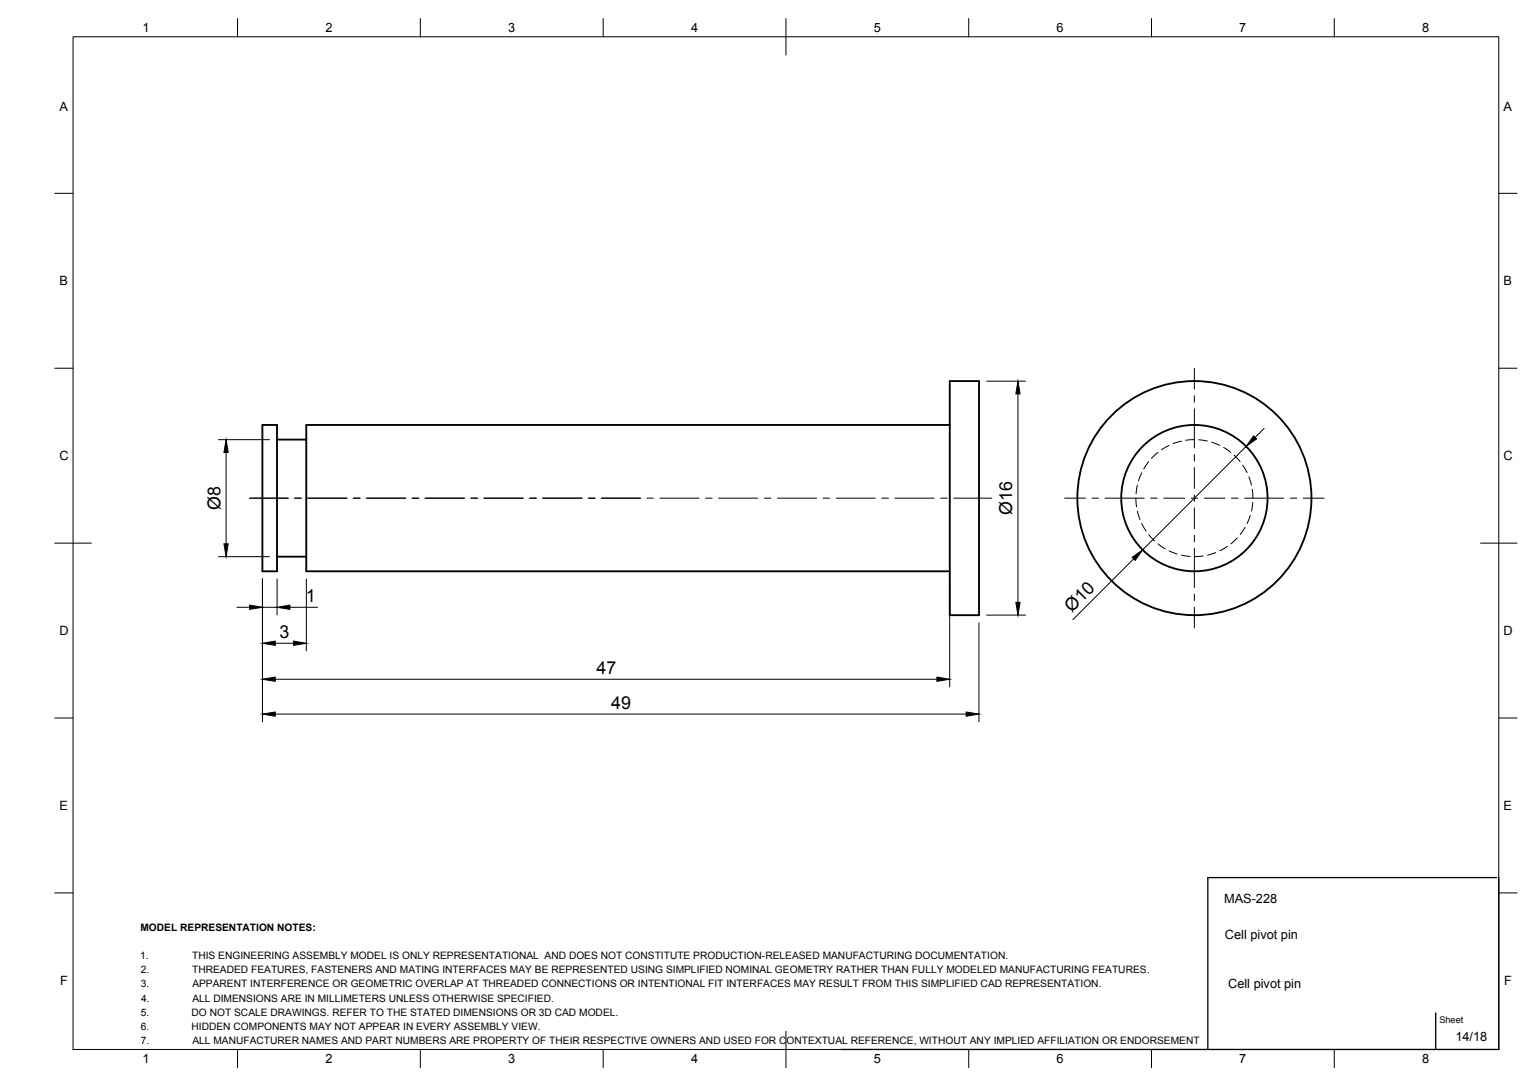
ISO-10303-21;
HEADER;
/* Generated by software containing ST-Developer
 * from STEP Tools, Inc. (www.steptools.com) 
 */

FILE_DESCRIPTION(
/* description */ ('Independent Peaucellier-Lipkin straight-line linkage. Radius arms 100
 mm, inversion-cell links 60 mm, crank radius and fixed-pivot spacing 
32 mm. Inversion constant 6400 mm squared, nominal output straight lin
e X=100 mm. Overhead bearing bridge clears the layered moving links. N
o accuracy or load rating assigned.'),
/* implementation_level */ '2;1');

FILE_NAME(
/* name */ 'Cell pivot pin.step',
/* time_stamp */ '2026-11-09T18:06:16-08:00',
/* author */ (''),
/* organization */ (''),
/* preprocessor_version */ 'ST-DEVELOPER v20.2',
/* originating_system */ 'Autodesk Translation Framework v15.17.0.0',
/* authorisation */ '');

FILE_SCHEMA (('AUTOMOTIVE_DESIGN { 1 0 10303 214 3 1 1 }'));
ENDSEC;

DATA;
#10=MECHANICAL_DESIGN_GEOMETRIC_PRESENTATION_REPRESENTATION('',(#295),#3581);
#261=SHAPE_REPRESENTATION_RELATIONSHIP('SRR','None',#3695,#278);
#278=ADVANCED_BREP_SHAPE_REPRESENTATION('',(#312),#3577);
#295=STYLED_ITEM('',(#3782),#312);
#312=MANIFOLD_SOLID_BREP('Body1',#1881);
#357=FACE_BOUND('',#667,.T.);
#358=FACE_BOUND('',#669,.T.);
#359=FACE_BOUND('',#672,.T.);
#412=PLANE('',#2257);
#413=PLANE('',#2259);
#414=PLANE('',#2263);
#415=PLANE('',#2268);
#416=PLANE('',#2270);
#513=FACE_OUTER_BOUND('',#665,.T.);
#514=FACE_OUTER_BOUND('',#666,.T.);
#515=FACE_OUTER_BOUND('',#668,.T.);
#516=FACE_OUTER_BOUND('',#670,.T.);
#517=FACE_OUTER_BOUND('',#671,.T.);
#518=FACE_OUTER_BOUND('',#673,.T.);
#519=FACE_OUTER_BOUND('',#674,.T.);
#520=FACE_OUTER_BOUND('',#675,.T.);
#521=FACE_OUTER_BOUND('',#676,.T.);
#665=EDGE_LOOP('',(#1636,#1637,#1638,#1639));
#666=EDGE_LOOP('',(#1640));
#667=EDGE_LOOP('',(#1641));
#668=EDGE_LOOP('',(#1642));
#669=EDGE_LOOP('',(#1643));
#670=EDGE_LOOP('',(#1644,#1645,#1646,#1647));
#671=EDGE_LOOP('',(#1648));
#672=EDGE_LOOP('',(#1649));
#673=EDGE_LOOP('',(#1650,#1651,#1652,#1653));
#674=EDGE_LOOP('',(#1654));
#675=EDGE_LOOP('',(#1655,#1656,#1657,#1658));
#676=EDGE_LOOP('',(#1659));
#777=LINE('',#3403,#875);
#778=LINE('',#3414,#876);
#779=LINE('',#3422,#877);
#780=LINE('',#3426,#878);
#875=VECTOR('',#2807,4.);
#876=VECTOR('',#2822,5.);
#877=VECTOR('',#2831,8.);
#878=VECTOR('',#2838,5.);
#969=CIRCLE('',#2255,4.);
#970=CIRCLE('',#2256,4.);
#971=CIRCLE('',#2258,5.);
#972=CIRCLE('',#2260,5.);
#973=CIRCLE('',#2262,5.);
#974=CIRCLE('',#2264,8.);
#975=CIRCLE('',#2265,5.);
#976=CIRCLE('',#2267,8.);
#1096=VERTEX_POINT('',#3400);
#1097=VERTEX_POINT('',#3402);
#1098=VERTEX_POINT('',#3406);
#1099=VERTEX_POINT('',#3409);
#1100=VERTEX_POINT('',#3412);
#1101=VERTEX_POINT('',#3416);
#1102=VERTEX_POINT('',#3418);
#1103=VERTEX_POINT('',#3421);
#1280=EDGE_CURVE('',#1096,#1096,#969,.T.);
#1281=EDGE_CURVE('',#1096,#1097,#777,.T.);
#1282=EDGE_CURVE('',#1097,#1097,#970,.T.);
#1283=EDGE_CURVE('',#1098,#1098,#971,.T.);
#1284=EDGE_CURVE('',#1099,#1099,#972,.T.);
#1285=EDGE_CURVE('',#1100,#1100,#973,.T.);
#1286=EDGE_CURVE('',#1100,#1099,#778,.T.);
#1287=EDGE_CURVE('',#1101,#1101,#974,.T.);
#1288=EDGE_CURVE('',#1102,#1102,#975,.T.);
#1289=EDGE_CURVE('',#1101,#1103,#779,.T.);
#1290=EDGE_CURVE('',#1103,#1103,#976,.T.);
#1291=EDGE_CURVE('',#1098,#1102,#780,.T.);
#1636=ORIENTED_EDGE('',*,*,#1280,.T.);
#1637=ORIENTED_EDGE('',*,*,#1281,.T.);
#1638=ORIENTED_EDGE('',*,*,#1282,.F.);
#1639=ORIENTED_EDGE('',*,*,#1281,.F.);
#1640=ORIENTED_EDGE('',*,*,#1283,.F.);
#1641=ORIENTED_EDGE('',*,*,#1280,.F.);
#1642=ORIENTED_EDGE('',*,*,#1284,.F.);
#1643=ORIENTED_EDGE('',*,*,#1282,.T.);
#1644=ORIENTED_EDGE('',*,*,#1285,.F.);
#1645=ORIENTED_EDGE('',*,*,#1286,.T.);
#1646=ORIENTED_EDGE('',*,*,#1284,.T.);
#1647=ORIENTED_EDGE('',*,*,#1286,.F.);
#1648=ORIENTED_EDGE('',*,*,#1287,.T.);
#1649=ORIENTED_EDGE('',*,*,#1288,.F.);
#1650=ORIENTED_EDGE('',*,*,#1287,.F.);
#1651=ORIENTED_EDGE('',*,*,#1289,.T.);
#1652=ORIENTED_EDGE('',*,*,#1290,.T.);
#1653=ORIENTED_EDGE('',*,*,#1289,.F.);
#1654=ORIENTED_EDGE('',*,*,#1290,.F.);
#1655=ORIENTED_EDGE('',*,*,#1283,.T.);
#1656=ORIENTED_EDGE('',*,*,#1291,.T.);
#1657=ORIENTED_EDGE('',*,*,#1288,.T.);
#1658=ORIENTED_EDGE('',*,*,#1291,.F.);
#1659=ORIENTED_EDGE('',*,*,#1285,.T.);
#1747=CYLINDRICAL_SURFACE('',#2254,4.);
#1748=CYLINDRICAL_SURFACE('',#2261,5.);
#1749=CYLINDRICAL_SURFACE('',#2266,8.);
#1750=CYLINDRICAL_SURFACE('',#2269,5.);
#1845=ADVANCED_FACE('',(#513),#1747,.T.);
#1846=ADVANCED_FACE('',(#514,#357),#412,.F.);
#1847=ADVANCED_FACE('',(#515,#358),#413,.F.);
#1848=ADVANCED_FACE('',(#516),#1748,.T.);
#1849=ADVANCED_FACE('',(#517,#359),#414,.T.);
#1850=ADVANCED_FACE('',(#518),#1749,.T.);
#1851=ADVANCED_FACE('',(#519),#415,.F.);
#1852=ADVANCED_FACE('',(#520),#1750,.T.);
#1853=ADVANCED_FACE('',(#521),#416,.T.);
#1881=CLOSED_SHELL('',(#1845,#1846,#1847,#1848,#1849,#1850,#1851,#1852,
#1853));
#2253=AXIS2_PLACEMENT_3D('',#3398,#2801,#2802);
#2254=AXIS2_PLACEMENT_3D('',#3399,#2803,#2804);
#2255=AXIS2_PLACEMENT_3D('',#3401,#2805,#2806);
#2256=AXIS2_PLACEMENT_3D('',#3404,#2808,#2809);
#2257=AXIS2_PLACEMENT_3D('',#3405,#2810,#2811);
#2258=AXIS2_PLACEMENT_3D('',#3407,#2812,#2813);
#2259=AXIS2_PLACEMENT_3D('',#3408,#2814,#2815);
#2260=AXIS2_PLACEMENT_3D('',#3410,#2816,#2817);
#2261=AXIS2_PLACEMENT_3D('',#3411,#2818,#2819);
#2262=AXIS2_PLACEMENT_3D('',#3413,#2820,#2821);
#2263=AXIS2_PLACEMENT_3D('',#3415,#2823,#2824);
#2264=AXIS2_PLACEMENT_3D('',#3417,#2825,#2826);
#2265=AXIS2_PLACEMENT_3D('',#3419,#2827,#2828);
#2266=AXIS2_PLACEMENT_3D('',#3420,#2829,#2830);
#2267=AXIS2_PLACEMENT_3D('',#3423,#2832,#2833);
#2268=AXIS2_PLACEMENT_3D('',#3424,#2834,#2835);
#2269=AXIS2_PLACEMENT_3D('',#3425,#2836,#2837);
#2270=AXIS2_PLACEMENT_3D('',#3427,#2839,#2840);
#2801=DIRECTION('axis',(0.,0.,1.));
#2802=DIRECTION('refdir',(1.,0.,0.));
#2803=DIRECTION('center_axis',(0.,0.,1.));
#2804=DIRECTION('ref_axis',(1.,0.,0.));
#2805=DIRECTION('center_axis',(0.,0.,1.));
#2806=DIRECTION('ref_axis',(1.,0.,0.));
#2807=DIRECTION('',(0.,0.,1.));
#2808=DIRECTION('center_axis',(0.,0.,1.));
#2809=DIRECTION('ref_axis',(1.,0.,0.));
#2810=DIRECTION('center_axis',(0.,0.,-1.));
#2811=DIRECTION('ref_axis',(-1.,0.,0.));
#2812=DIRECTION('center_axis',(0.,0.,-1.));
#2813=DIRECTION('ref_axis',(1.,0.,0.));
#2814=DIRECTION('center_axis',(0.,0.,1.));
#2815=DIRECTION('ref_axis',(1.,0.,0.));
#2816=DIRECTION('center_axis',(0.,0.,1.));
#2817=DIRECTION('ref_axis',(1.,0.,0.));
#2818=DIRECTION('center_axis',(0.,0.,1.));
#2819=DIRECTION('ref_axis',(1.,0.,0.));
#2820=DIRECTION('center_axis',(0.,0.,1.));
#2821=DIRECTION('ref_axis',(1.,0.,0.));
#2822=DIRECTION('',(0.,0.,-1.));
#2823=DIRECTION('center_axis',(0.,0.,1.));
#2824=DIRECTION('ref_axis',(1.,0.,0.));
#2825=DIRECTION('center_axis',(0.,0.,1.));
#2826=DIRECTION('ref_axis',(1.,0.,0.));
#2827=DIRECTION('center_axis',(0.,0.,1.));
#2828=DIRECTION('ref_axis',(1.,0.,0.));
#2829=DIRECTION('center_axis',(0.,0.,1.));
#2830=DIRECTION('ref_axis',(1.,0.,0.));
#2831=DIRECTION('',(0.,0.,-1.));
#2832=DIRECTION('center_axis',(0.,0.,1.));
#2833=DIRECTION('ref_axis',(1.,0.,0.));
#2834=DIRECTION('center_axis',(0.,0.,1.));
#2835=DIRECTION('ref_axis',(1.,0.,0.));
#2836=DIRECTION('center_axis',(0.,0.,1.));
#2837=DIRECTION('ref_axis',(1.,0.,0.));
#2838=DIRECTION('',(0.,0.,-1.));
#2839=DIRECTION('center_axis',(0.,0.,1.));
#2840=DIRECTION('ref_axis',(1.,0.,0.));
#3398=CARTESIAN_POINT('',(0.,0.,0.));
#3399=CARTESIAN_POINT('Origin',(0.,0.,45.));
#3400=CARTESIAN_POINT('',(-4.,-4.89858719658941E-16,44.));
#3401=CARTESIAN_POINT('Origin',(0.,0.,44.));
#3402=CARTESIAN_POINT('',(-4.,-4.89858719658941E-16,46.));
#3403=CARTESIAN_POINT('',(-4.,-4.89858719658941E-16,45.));
#3404=CARTESIAN_POINT('Origin',(0.,0.,46.));
#3405=CARTESIAN_POINT('Origin',(8.,0.,44.));
#3406=CARTESIAN_POINT('',(-5.,6.12323399573677E-16,44.));
#3407=CARTESIAN_POINT('Origin',(0.,0.,44.));
#3408=CARTESIAN_POINT('Origin',(4.,0.,46.));
#3409=CARTESIAN_POINT('',(-5.,-6.12323399573677E-16,46.));
#3410=CARTESIAN_POINT('Origin',(0.,0.,46.));
#3411=CARTESIAN_POINT('Origin',(0.,0.,0.));
#3412=CARTESIAN_POINT('',(-5.,-6.12323399573677E-16,47.));
#3413=CARTESIAN_POINT('Origin',(0.,0.,47.));
#3414=CARTESIAN_POINT('',(-5.,-6.12323399573677E-16,0.));
#3415=CARTESIAN_POINT('Origin',(0.,0.,0.));
#3416=CARTESIAN_POINT('',(-8.,-9.79717439317883E-16,0.));
#3417=CARTESIAN_POINT('Origin',(0.,0.,0.));
#3418=CARTESIAN_POINT('',(-5.,-6.12323399573677E-16,0.));
#3419=CARTESIAN_POINT('Origin',(0.,0.,0.));
#3420=CARTESIAN_POINT('Origin',(0.,0.,-2.));
#3421=CARTESIAN_POINT('',(-8.,-9.79717439317883E-16,-2.));
#3422=CARTESIAN_POINT('',(-8.,-9.79717439317883E-16,-2.));
#3423=CARTESIAN_POINT('Origin',(0.,0.,-2.));
#3424=CARTESIAN_POINT('Origin',(0.,0.,-2.));
#3425=CARTESIAN_POINT('Origin',(0.,0.,0.));
#3426=CARTESIAN_POINT('',(-5.,-6.12323399573677E-16,0.));
#3427=CARTESIAN_POINT('Origin',(0.,0.,47.));
#3558=UNCERTAINTY_MEASURE_WITH_UNIT(LENGTH_MEASURE(0.01),#3582,
'DISTANCE_ACCURACY_VALUE',
'Maximum model space distance between geometric entities at asserted c
onnectivities');
#3562=UNCERTAINTY_MEASURE_WITH_UNIT(LENGTH_MEASURE(0.01),#3582,
'DISTANCE_ACCURACY_VALUE',
'Maximum model space distance between geometric entities at asserted c
onnectivities');
#3577=(
GEOMETRIC_REPRESENTATION_CONTEXT(3)
GLOBAL_UNCERTAINTY_ASSIGNED_CONTEXT((#3558))
GLOBAL_UNIT_ASSIGNED_CONTEXT((#3582,#3584,#3585))
REPRESENTATION_CONTEXT('','3D')
);
#3581=(
GEOMETRIC_REPRESENTATION_CONTEXT(3)
GLOBAL_UNCERTAINTY_ASSIGNED_CONTEXT((#3562))
GLOBAL_UNIT_ASSIGNED_CONTEXT((#3582,#3584,#3585))
REPRESENTATION_CONTEXT('','3D')
);
#3582=(
LENGTH_UNIT()
NAMED_UNIT(*)
SI_UNIT(.MILLI.,.METRE.)
);
#3584=(
NAMED_UNIT(*)
PLANE_ANGLE_UNIT()
SI_UNIT($,.RADIAN.)
);
#3585=(
NAMED_UNIT(*)
SI_UNIT($,.STERADIAN.)
SOLID_ANGLE_UNIT()
);
#3600=SHAPE_DEFINITION_REPRESENTATION(#3618,#3695);
#3618=PRODUCT_DEFINITION_SHAPE('',$,#3714);
#3695=SHAPE_REPRESENTATION('',(#2253),#3577);
#3699=PRODUCT_DEFINITION_CONTEXT('part definition',#3755,'design');
#3714=PRODUCT_DEFINITION('Cell pivot pin','Cell pivot pin',#3732,#3699);
#3732=PRODUCT_DEFINITION_FORMATION('',$,#3771);
#3755=APPLICATION_CONTEXT(
'Core Data for Automotive Mechanical Design Process');
#3756=PRODUCT_CONTEXT('part definition',#3755,'mechanical');
#3771=PRODUCT('Cell pivot pin','Cell pivot pin',$,(#3756));
#3782=PRESENTATION_STYLE_ASSIGNMENT((#3795));
#3795=SURFACE_STYLE_USAGE(.BOTH.,#3808);
#3808=SURFACE_SIDE_STYLE('',(#3821));
#3821=SURFACE_STYLE_FILL_AREA(#3834);
#3834=FILL_AREA_STYLE('Pivot gray',(#3847));
#3847=FILL_AREA_STYLE_COLOUR('Pivot gray',#3860);
#3860=COLOUR_RGB('Pivot gray',0.407843137254902,0.447058823529412,0.498039215686275);
ENDSEC;
END-ISO-10303-21;
